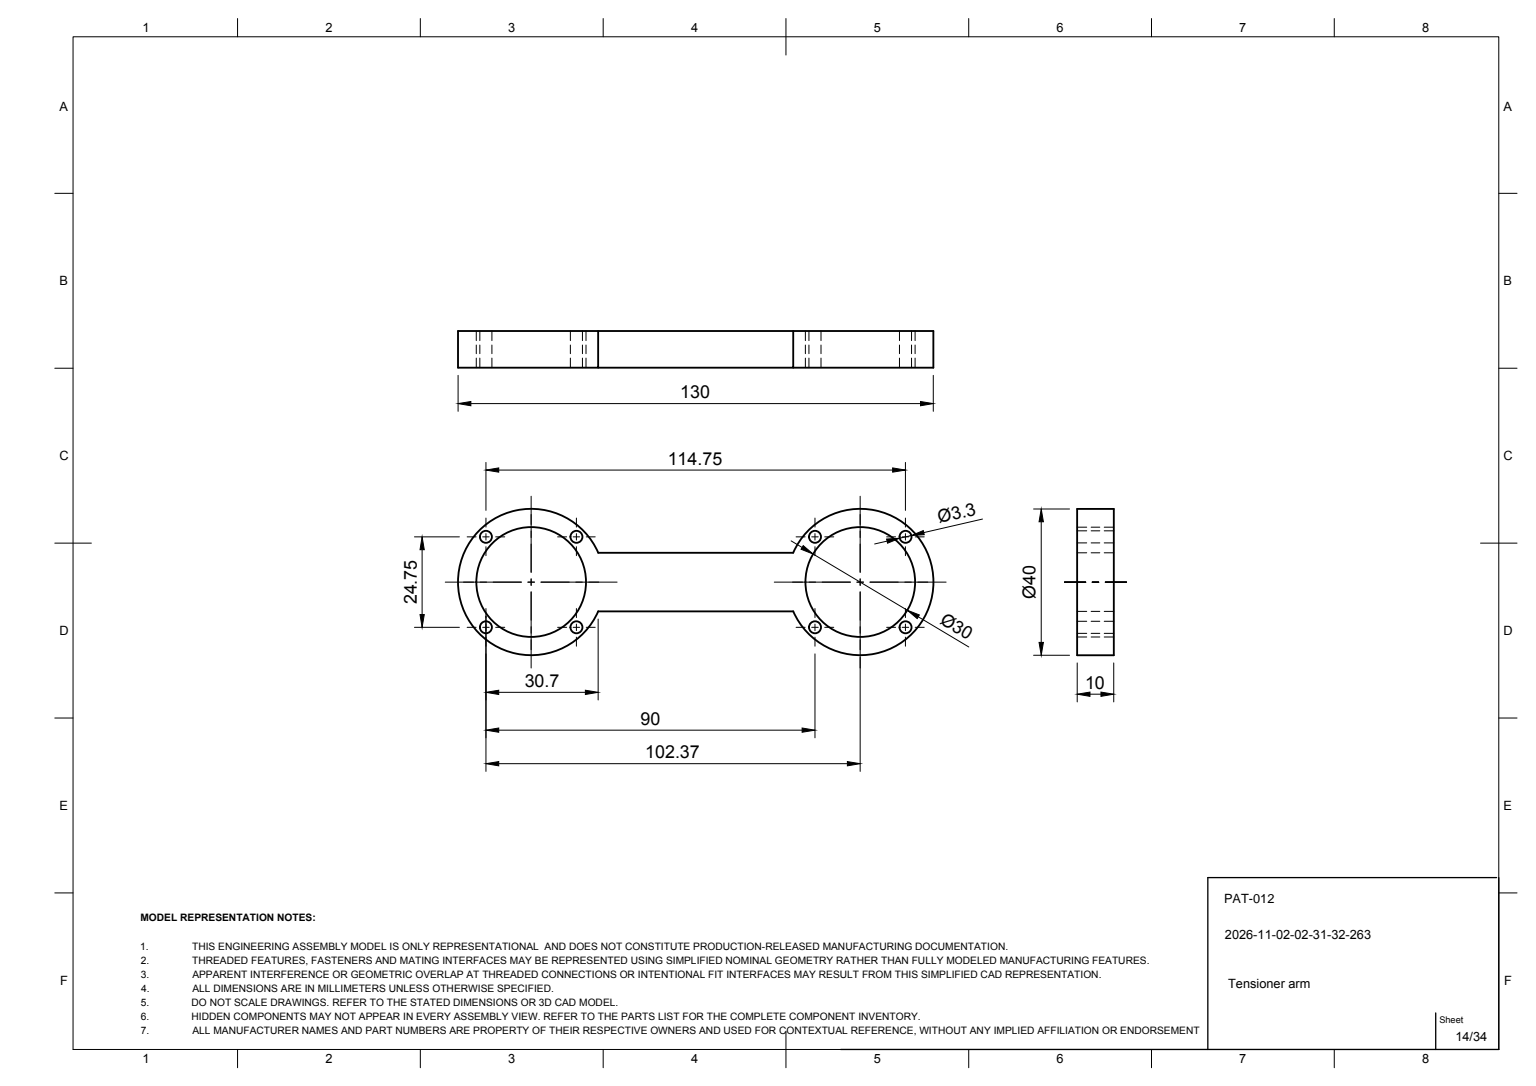
ISO-10303-21;
HEADER;
/* Generated by software containing ST-Developer
 * from STEP Tools, Inc. (www.steptools.com) 
 */

FILE_DESCRIPTION(
/* description */ ('Belt tensioner idler arm'),
/* implementation_level */ '2;1');

FILE_NAME(
/* name */ 'Tensioner arm.step',
/* time_stamp */ '2026-10-28T03:22:15-07:00',
/* author */ (''),
/* organization */ (''),
/* preprocessor_version */ 'ST-DEVELOPER v20.2',
/* originating_system */ 'Autodesk Translation Framework v15.17.0.0',
/* authorisation */ '');

FILE_SCHEMA (('AUTOMOTIVE_DESIGN { 1 0 10303 214 3 1 1 }'));
ENDSEC;

DATA;
#10=MECHANICAL_DESIGN_GEOMETRIC_PRESENTATION_REPRESENTATION('',(#459),#12779);
#391=SHAPE_REPRESENTATION_RELATIONSHIP('SRR','None',#12938,#425);
#425=ADVANCED_BREP_SHAPE_REPRESENTATION('',(#499),#12755);
#459=STYLED_ITEM('',(#13177),#499);
#499=MANIFOLD_SOLID_BREP('Body1',#6195);
#562=FACE_BOUND('',#1371,.T.);
#563=FACE_BOUND('',#1372,.T.);
#564=FACE_BOUND('',#1373,.T.);
#565=FACE_BOUND('',#1374,.T.);
#566=FACE_BOUND('',#1375,.T.);
#567=FACE_BOUND('',#1376,.T.);
#568=FACE_BOUND('',#1377,.T.);
#569=FACE_BOUND('',#1378,.T.);
#570=FACE_BOUND('',#1379,.T.);
#571=FACE_BOUND('',#1380,.T.);
#572=FACE_BOUND('',#1384,.T.);
#573=FACE_BOUND('',#1385,.T.);
#574=FACE_BOUND('',#1386,.T.);
#575=FACE_BOUND('',#1387,.T.);
#576=FACE_BOUND('',#1388,.T.);
#577=FACE_BOUND('',#1389,.T.);
#578=FACE_BOUND('',#1390,.T.);
#579=FACE_BOUND('',#1391,.T.);
#580=FACE_BOUND('',#1392,.T.);
#581=FACE_BOUND('',#1393,.T.);
#740=PLANE('',#6843);
#741=PLANE('',#6844);
#742=PLANE('',#6846);
#743=PLANE('',#6849);
#956=FACE_OUTER_BOUND('',#1358,.T.);
#957=FACE_OUTER_BOUND('',#1359,.T.);
#958=FACE_OUTER_BOUND('',#1360,.T.);
#959=FACE_OUTER_BOUND('',#1361,.T.);
#960=FACE_OUTER_BOUND('',#1362,.T.);
#961=FACE_OUTER_BOUND('',#1363,.T.);
#962=FACE_OUTER_BOUND('',#1364,.T.);
#963=FACE_OUTER_BOUND('',#1365,.T.);
#964=FACE_OUTER_BOUND('',#1366,.T.);
#965=FACE_OUTER_BOUND('',#1367,.T.);
#966=FACE_OUTER_BOUND('',#1368,.T.);
#967=FACE_OUTER_BOUND('',#1369,.T.);
#968=FACE_OUTER_BOUND('',#1370,.T.);
#969=FACE_OUTER_BOUND('',#1381,.T.);
#970=FACE_OUTER_BOUND('',#1382,.T.);
#971=FACE_OUTER_BOUND('',#1383,.T.);
#1358=EDGE_LOOP('',(#4554,#4555,#4556,#4557));
#1359=EDGE_LOOP('',(#4558,#4559,#4560,#4561));
#1360=EDGE_LOOP('',(#4562,#4563,#4564,#4565));
#1361=EDGE_LOOP('',(#4566,#4567,#4568,#4569));
#1362=EDGE_LOOP('',(#4570,#4571,#4572,#4573));
#1363=EDGE_LOOP('',(#4574,#4575,#4576,#4577));
#1364=EDGE_LOOP('',(#4578,#4579,#4580,#4581));
#1365=EDGE_LOOP('',(#4582,#4583,#4584,#4585));
#1366=EDGE_LOOP('',(#4586,#4587,#4588,#4589));
#1367=EDGE_LOOP('',(#4590,#4591,#4592,#4593));
#1368=EDGE_LOOP('',(#4594,#4595,#4596,#4597));
#1369=EDGE_LOOP('',(#4598,#4599,#4600,#4601));
#1370=EDGE_LOOP('',(#4602,#4603,#4604,#4605));
#1371=EDGE_LOOP('',(#4606));
#1372=EDGE_LOOP('',(#4607));
#1373=EDGE_LOOP('',(#4608));
#1374=EDGE_LOOP('',(#4609));
#1375=EDGE_LOOP('',(#4610));
#1376=EDGE_LOOP('',(#4611));
#1377=EDGE_LOOP('',(#4612));
#1378=EDGE_LOOP('',(#4613));
#1379=EDGE_LOOP('',(#4614));
#1380=EDGE_LOOP('',(#4615));
#1381=EDGE_LOOP('',(#4616,#4617,#4618,#4619));
#1382=EDGE_LOOP('',(#4620,#4621,#4622,#4623));
#1383=EDGE_LOOP('',(#4624,#4625,#4626,#4627));
#1384=EDGE_LOOP('',(#4628));
#1385=EDGE_LOOP('',(#4629));
#1386=EDGE_LOOP('',(#4630));
#1387=EDGE_LOOP('',(#4631));
#1388=EDGE_LOOP('',(#4632));
#1389=EDGE_LOOP('',(#4633));
#1390=EDGE_LOOP('',(#4634));
#1391=EDGE_LOOP('',(#4635));
#1392=EDGE_LOOP('',(#4636));
#1393=EDGE_LOOP('',(#4637));
#1843=LINE('',#10693,#2192);
#1844=LINE('',#10699,#2193);
#1845=LINE('',#10705,#2194);
#1846=LINE('',#10711,#2195);
#1847=LINE('',#10717,#2196);
#1848=LINE('',#10723,#2197);
#1849=LINE('',#10729,#2198);
#1850=LINE('',#10735,#2199);
#1851=LINE('',#10741,#2200);
#1852=LINE('',#10747,#2201);
#1853=LINE('',#10752,#2202);
#1854=LINE('',#10756,#2203);
#1855=LINE('',#10760,#2204);
#1856=LINE('',#10762,#2205);
#1857=LINE('',#10763,#2206);
#1858=LINE('',#10766,#2207);
#1859=LINE('',#10770,#2208);
#1860=LINE('',#10771,#2209);
#2192=VECTOR('',#7989,0.165);
#2193=VECTOR('',#7996,0.165);
#2194=VECTOR('',#8003,0.164999999999999);
#2195=VECTOR('',#8010,0.164999999999999);
#2196=VECTOR('',#8017,0.165);
#2197=VECTOR('',#8024,0.165);
#2198=VECTOR('',#8031,0.165);
#2199=VECTOR('',#8038,0.165);
#2200=VECTOR('',#8045,1.5);
#2201=VECTOR('',#8052,1.5);
#2202=VECTOR('',#8057,1.);
#2203=VECTOR('',#8060,1.);
#2204=VECTOR('',#8065,1.);
#2205=VECTOR('',#8066,1.);
#2206=VECTOR('',#8067,1.);
#2207=VECTOR('',#8070,1.);
#2208=VECTOR('',#8075,1.);
#2209=VECTOR('',#8076,1.);
#2478=CIRCLE('',#6811,0.165);
#2479=CIRCLE('',#6812,0.165);
#2480=CIRCLE('',#6814,0.165);
#2481=CIRCLE('',#6815,0.165);
#2482=CIRCLE('',#6817,0.164999999999999);
#2483=CIRCLE('',#6818,0.164999999999999);
#2484=CIRCLE('',#6820,0.164999999999999);
#2485=CIRCLE('',#6821,0.164999999999999);
#2486=CIRCLE('',#6823,0.165);
#2487=CIRCLE('',#6824,0.165);
#2488=CIRCLE('',#6826,0.165);
#2489=CIRCLE('',#6827,0.165);
#2490=CIRCLE('',#6829,0.165);
#2491=CIRCLE('',#6830,0.165);
#2492=CIRCLE('',#6832,0.165);
#2493=CIRCLE('',#6833,0.165);
#2494=CIRCLE('',#6835,1.5);
#2495=CIRCLE('',#6836,1.5);
#2496=CIRCLE('',#6838,1.5);
#2497=CIRCLE('',#6839,1.5);
#2498=CIRCLE('',#6841,2.);
#2499=CIRCLE('',#6842,2.);
#2500=CIRCLE('',#6845,2.);
#2501=CIRCLE('',#6848,2.);
#2919=VERTEX_POINT('',#10690);
#2920=VERTEX_POINT('',#10692);
#2921=VERTEX_POINT('',#10696);
#2922=VERTEX_POINT('',#10698);
#2923=VERTEX_POINT('',#10702);
#2924=VERTEX_POINT('',#10704);
#2925=VERTEX_POINT('',#10708);
#2926=VERTEX_POINT('',#10710);
#2927=VERTEX_POINT('',#10714);
#2928=VERTEX_POINT('',#10716);
#2929=VERTEX_POINT('',#10720);
#2930=VERTEX_POINT('',#10722);
#2931=VERTEX_POINT('',#10726);
#2932=VERTEX_POINT('',#10728);
#2933=VERTEX_POINT('',#10732);
#2934=VERTEX_POINT('',#10734);
#2935=VERTEX_POINT('',#10738);
#2936=VERTEX_POINT('',#10740);
#2937=VERTEX_POINT('',#10744);
#2938=VERTEX_POINT('',#10746);
#2939=VERTEX_POINT('',#10750);
#2940=VERTEX_POINT('',#10751);
#2941=VERTEX_POINT('',#10753);
#2942=VERTEX_POINT('',#10755);
#2943=VERTEX_POINT('',#10759);
#2944=VERTEX_POINT('',#10761);
#2945=VERTEX_POINT('',#10765);
#2946=VERTEX_POINT('',#10769);
#3532=EDGE_CURVE('',#2919,#2919,#2478,.T.);
#3533=EDGE_CURVE('',#2919,#2920,#1843,.T.);
#3534=EDGE_CURVE('',#2920,#2920,#2479,.T.);
#3535=EDGE_CURVE('',#2921,#2921,#2480,.T.);
#3536=EDGE_CURVE('',#2921,#2922,#1844,.T.);
#3537=EDGE_CURVE('',#2922,#2922,#2481,.T.);
#3538=EDGE_CURVE('',#2923,#2923,#2482,.T.);
#3539=EDGE_CURVE('',#2923,#2924,#1845,.T.);
#3540=EDGE_CURVE('',#2924,#2924,#2483,.T.);
#3541=EDGE_CURVE('',#2925,#2925,#2484,.T.);
#3542=EDGE_CURVE('',#2925,#2926,#1846,.T.);
#3543=EDGE_CURVE('',#2926,#2926,#2485,.T.);
#3544=EDGE_CURVE('',#2927,#2927,#2486,.T.);
#3545=EDGE_CURVE('',#2927,#2928,#1847,.T.);
#3546=EDGE_CURVE('',#2928,#2928,#2487,.T.);
#3547=EDGE_CURVE('',#2929,#2929,#2488,.T.);
#3548=EDGE_CURVE('',#2929,#2930,#1848,.T.);
#3549=EDGE_CURVE('',#2930,#2930,#2489,.T.);
#3550=EDGE_CURVE('',#2931,#2931,#2490,.T.);
#3551=EDGE_CURVE('',#2931,#2932,#1849,.T.);
#3552=EDGE_CURVE('',#2932,#2932,#2491,.T.);
#3553=EDGE_CURVE('',#2933,#2933,#2492,.T.);
#3554=EDGE_CURVE('',#2933,#2934,#1850,.T.);
#3555=EDGE_CURVE('',#2934,#2934,#2493,.T.);
#3556=EDGE_CURVE('',#2935,#2935,#2494,.T.);
#3557=EDGE_CURVE('',#2935,#2936,#1851,.T.);
#3558=EDGE_CURVE('',#2936,#2936,#2495,.T.);
#3559=EDGE_CURVE('',#2937,#2937,#2496,.T.);
#3560=EDGE_CURVE('',#2937,#2938,#1852,.T.);
#3561=EDGE_CURVE('',#2938,#2938,#2497,.T.);
#3562=EDGE_CURVE('',#2939,#2940,#1853,.T.);
#3563=EDGE_CURVE('',#2941,#2939,#2498,.T.);
#3564=EDGE_CURVE('',#2942,#2941,#1854,.T.);
#3565=EDGE_CURVE('',#2942,#2940,#2499,.T.);
#3566=EDGE_CURVE('',#2940,#2943,#1855,.T.);
#3567=EDGE_CURVE('',#2944,#2943,#1856,.T.);
#3568=EDGE_CURVE('',#2939,#2944,#1857,.T.);
#3569=EDGE_CURVE('',#2945,#2942,#1858,.T.);
#3570=EDGE_CURVE('',#2943,#2945,#2500,.T.);
#3571=EDGE_CURVE('',#2946,#2941,#1859,.T.);
#3572=EDGE_CURVE('',#2945,#2946,#1860,.T.);
#3573=EDGE_CURVE('',#2944,#2946,#2501,.T.);
#4554=ORIENTED_EDGE('',*,*,#3532,.F.);
#4555=ORIENTED_EDGE('',*,*,#3533,.T.);
#4556=ORIENTED_EDGE('',*,*,#3534,.F.);
#4557=ORIENTED_EDGE('',*,*,#3533,.F.);
#4558=ORIENTED_EDGE('',*,*,#3535,.F.);
#4559=ORIENTED_EDGE('',*,*,#3536,.T.);
#4560=ORIENTED_EDGE('',*,*,#3537,.F.);
#4561=ORIENTED_EDGE('',*,*,#3536,.F.);
#4562=ORIENTED_EDGE('',*,*,#3538,.F.);
#4563=ORIENTED_EDGE('',*,*,#3539,.T.);
#4564=ORIENTED_EDGE('',*,*,#3540,.F.);
#4565=ORIENTED_EDGE('',*,*,#3539,.F.);
#4566=ORIENTED_EDGE('',*,*,#3541,.F.);
#4567=ORIENTED_EDGE('',*,*,#3542,.T.);
#4568=ORIENTED_EDGE('',*,*,#3543,.F.);
#4569=ORIENTED_EDGE('',*,*,#3542,.F.);
#4570=ORIENTED_EDGE('',*,*,#3544,.F.);
#4571=ORIENTED_EDGE('',*,*,#3545,.T.);
#4572=ORIENTED_EDGE('',*,*,#3546,.F.);
#4573=ORIENTED_EDGE('',*,*,#3545,.F.);
#4574=ORIENTED_EDGE('',*,*,#3547,.F.);
#4575=ORIENTED_EDGE('',*,*,#3548,.T.);
#4576=ORIENTED_EDGE('',*,*,#3549,.F.);
#4577=ORIENTED_EDGE('',*,*,#3548,.F.);
#4578=ORIENTED_EDGE('',*,*,#3550,.F.);
#4579=ORIENTED_EDGE('',*,*,#3551,.T.);
#4580=ORIENTED_EDGE('',*,*,#3552,.F.);
#4581=ORIENTED_EDGE('',*,*,#3551,.F.);
#4582=ORIENTED_EDGE('',*,*,#3553,.F.);
#4583=ORIENTED_EDGE('',*,*,#3554,.T.);
#4584=ORIENTED_EDGE('',*,*,#3555,.F.);
#4585=ORIENTED_EDGE('',*,*,#3554,.F.);
#4586=ORIENTED_EDGE('',*,*,#3556,.F.);
#4587=ORIENTED_EDGE('',*,*,#3557,.T.);
#4588=ORIENTED_EDGE('',*,*,#3558,.F.);
#4589=ORIENTED_EDGE('',*,*,#3557,.F.);
#4590=ORIENTED_EDGE('',*,*,#3559,.F.);
#4591=ORIENTED_EDGE('',*,*,#3560,.T.);
#4592=ORIENTED_EDGE('',*,*,#3561,.F.);
#4593=ORIENTED_EDGE('',*,*,#3560,.F.);
#4594=ORIENTED_EDGE('',*,*,#3562,.F.);
#4595=ORIENTED_EDGE('',*,*,#3563,.F.);
#4596=ORIENTED_EDGE('',*,*,#3564,.F.);
#4597=ORIENTED_EDGE('',*,*,#3565,.T.);
#4598=ORIENTED_EDGE('',*,*,#3562,.T.);
#4599=ORIENTED_EDGE('',*,*,#3566,.T.);
#4600=ORIENTED_EDGE('',*,*,#3567,.F.);
#4601=ORIENTED_EDGE('',*,*,#3568,.F.);
#4602=ORIENTED_EDGE('',*,*,#3565,.F.);
#4603=ORIENTED_EDGE('',*,*,#3569,.F.);
#4604=ORIENTED_EDGE('',*,*,#3570,.F.);
#4605=ORIENTED_EDGE('',*,*,#3566,.F.);
#4606=ORIENTED_EDGE('',*,*,#3544,.T.);
#4607=ORIENTED_EDGE('',*,*,#3547,.T.);
#4608=ORIENTED_EDGE('',*,*,#3550,.T.);
#4609=ORIENTED_EDGE('',*,*,#3553,.T.);
#4610=ORIENTED_EDGE('',*,*,#3556,.T.);
#4611=ORIENTED_EDGE('',*,*,#3559,.T.);
#4612=ORIENTED_EDGE('',*,*,#3541,.T.);
#4613=ORIENTED_EDGE('',*,*,#3538,.T.);
#4614=ORIENTED_EDGE('',*,*,#3535,.T.);
#4615=ORIENTED_EDGE('',*,*,#3532,.T.);
#4616=ORIENTED_EDGE('',*,*,#3564,.T.);
#4617=ORIENTED_EDGE('',*,*,#3571,.F.);
#4618=ORIENTED_EDGE('',*,*,#3572,.F.);
#4619=ORIENTED_EDGE('',*,*,#3569,.T.);
#4620=ORIENTED_EDGE('',*,*,#3567,.T.);
#4621=ORIENTED_EDGE('',*,*,#3570,.T.);
#4622=ORIENTED_EDGE('',*,*,#3572,.T.);
#4623=ORIENTED_EDGE('',*,*,#3573,.F.);
#4624=ORIENTED_EDGE('',*,*,#3568,.T.);
#4625=ORIENTED_EDGE('',*,*,#3573,.T.);
#4626=ORIENTED_EDGE('',*,*,#3571,.T.);
#4627=ORIENTED_EDGE('',*,*,#3563,.T.);
#4628=ORIENTED_EDGE('',*,*,#3546,.T.);
#4629=ORIENTED_EDGE('',*,*,#3549,.T.);
#4630=ORIENTED_EDGE('',*,*,#3552,.T.);
#4631=ORIENTED_EDGE('',*,*,#3555,.T.);
#4632=ORIENTED_EDGE('',*,*,#3558,.T.);
#4633=ORIENTED_EDGE('',*,*,#3561,.T.);
#4634=ORIENTED_EDGE('',*,*,#3543,.T.);
#4635=ORIENTED_EDGE('',*,*,#3540,.T.);
#4636=ORIENTED_EDGE('',*,*,#3537,.T.);
#4637=ORIENTED_EDGE('',*,*,#3534,.T.);
#5692=CYLINDRICAL_SURFACE('',#6810,0.165);
#5693=CYLINDRICAL_SURFACE('',#6813,0.165);
#5694=CYLINDRICAL_SURFACE('',#6816,0.164999999999999);
#5695=CYLINDRICAL_SURFACE('',#6819,0.164999999999999);
#5696=CYLINDRICAL_SURFACE('',#6822,0.165);
#5697=CYLINDRICAL_SURFACE('',#6825,0.165);
#5698=CYLINDRICAL_SURFACE('',#6828,0.165);
#5699=CYLINDRICAL_SURFACE('',#6831,0.165);
#5700=CYLINDRICAL_SURFACE('',#6834,1.5);
#5701=CYLINDRICAL_SURFACE('',#6837,1.5);
#5702=CYLINDRICAL_SURFACE('',#6840,2.);
#5703=CYLINDRICAL_SURFACE('',#6847,2.);
#5933=ADVANCED_FACE('',(#956),#5692,.F.);
#5934=ADVANCED_FACE('',(#957),#5693,.F.);
#5935=ADVANCED_FACE('',(#958),#5694,.F.);
#5936=ADVANCED_FACE('',(#959),#5695,.F.);
#5937=ADVANCED_FACE('',(#960),#5696,.F.);
#5938=ADVANCED_FACE('',(#961),#5697,.F.);
#5939=ADVANCED_FACE('',(#962),#5698,.F.);
#5940=ADVANCED_FACE('',(#963),#5699,.F.);
#5941=ADVANCED_FACE('',(#964),#5700,.F.);
#5942=ADVANCED_FACE('',(#965),#5701,.F.);
#5943=ADVANCED_FACE('',(#966),#5702,.T.);
#5944=ADVANCED_FACE('',(#967),#740,.T.);
#5945=ADVANCED_FACE('',(#968,#562,#563,#564,#565,#566,#567,#568,#569,#570,
#571),#741,.F.);
#5946=ADVANCED_FACE('',(#969),#742,.T.);
#5947=ADVANCED_FACE('',(#970),#5703,.T.);
#5948=ADVANCED_FACE('',(#971,#572,#573,#574,#575,#576,#577,#578,#579,#580,
#581),#743,.T.);
#6195=CLOSED_SHELL('',(#5933,#5934,#5935,#5936,#5937,#5938,#5939,#5940,
#5941,#5942,#5943,#5944,#5945,#5946,#5947,#5948));
#6809=AXIS2_PLACEMENT_3D('',#10688,#7983,#7984);
#6810=AXIS2_PLACEMENT_3D('',#10689,#7985,#7986);
#6811=AXIS2_PLACEMENT_3D('',#10691,#7987,#7988);
#6812=AXIS2_PLACEMENT_3D('',#10694,#7990,#7991);
#6813=AXIS2_PLACEMENT_3D('',#10695,#7992,#7993);
#6814=AXIS2_PLACEMENT_3D('',#10697,#7994,#7995);
#6815=AXIS2_PLACEMENT_3D('',#10700,#7997,#7998);
#6816=AXIS2_PLACEMENT_3D('',#10701,#7999,#8000);
#6817=AXIS2_PLACEMENT_3D('',#10703,#8001,#8002);
#6818=AXIS2_PLACEMENT_3D('',#10706,#8004,#8005);
#6819=AXIS2_PLACEMENT_3D('',#10707,#8006,#8007);
#6820=AXIS2_PLACEMENT_3D('',#10709,#8008,#8009);
#6821=AXIS2_PLACEMENT_3D('',#10712,#8011,#8012);
#6822=AXIS2_PLACEMENT_3D('',#10713,#8013,#8014);
#6823=AXIS2_PLACEMENT_3D('',#10715,#8015,#8016);
#6824=AXIS2_PLACEMENT_3D('',#10718,#8018,#8019);
#6825=AXIS2_PLACEMENT_3D('',#10719,#8020,#8021);
#6826=AXIS2_PLACEMENT_3D('',#10721,#8022,#8023);
#6827=AXIS2_PLACEMENT_3D('',#10724,#8025,#8026);
#6828=AXIS2_PLACEMENT_3D('',#10725,#8027,#8028);
#6829=AXIS2_PLACEMENT_3D('',#10727,#8029,#8030);
#6830=AXIS2_PLACEMENT_3D('',#10730,#8032,#8033);
#6831=AXIS2_PLACEMENT_3D('',#10731,#8034,#8035);
#6832=AXIS2_PLACEMENT_3D('',#10733,#8036,#8037);
#6833=AXIS2_PLACEMENT_3D('',#10736,#8039,#8040);
#6834=AXIS2_PLACEMENT_3D('',#10737,#8041,#8042);
#6835=AXIS2_PLACEMENT_3D('',#10739,#8043,#8044);
#6836=AXIS2_PLACEMENT_3D('',#10742,#8046,#8047);
#6837=AXIS2_PLACEMENT_3D('',#10743,#8048,#8049);
#6838=AXIS2_PLACEMENT_3D('',#10745,#8050,#8051);
#6839=AXIS2_PLACEMENT_3D('',#10748,#8053,#8054);
#6840=AXIS2_PLACEMENT_3D('',#10749,#8055,#8056);
#6841=AXIS2_PLACEMENT_3D('',#10754,#8058,#8059);
#6842=AXIS2_PLACEMENT_3D('',#10757,#8061,#8062);
#6843=AXIS2_PLACEMENT_3D('',#10758,#8063,#8064);
#6844=AXIS2_PLACEMENT_3D('',#10764,#8068,#8069);
#6845=AXIS2_PLACEMENT_3D('',#10767,#8071,#8072);
#6846=AXIS2_PLACEMENT_3D('',#10768,#8073,#8074);
#6847=AXIS2_PLACEMENT_3D('',#10772,#8077,#8078);
#6848=AXIS2_PLACEMENT_3D('',#10773,#8079,#8080);
#6849=AXIS2_PLACEMENT_3D('',#10774,#8081,#8082);
#7983=DIRECTION('axis',(0.,0.,1.));
#7984=DIRECTION('refdir',(1.,0.,0.));
#7985=DIRECTION('center_axis',(0.,0.,1.));
#7986=DIRECTION('ref_axis',(1.,0.,0.));
#7987=DIRECTION('center_axis',(0.,0.,1.));
#7988=DIRECTION('ref_axis',(1.,0.,0.));
#7989=DIRECTION('',(0.,0.,1.));
#7990=DIRECTION('center_axis',(0.,0.,-1.));
#7991=DIRECTION('ref_axis',(1.,0.,0.));
#7992=DIRECTION('center_axis',(0.,0.,1.));
#7993=DIRECTION('ref_axis',(1.,0.,0.));
#7994=DIRECTION('center_axis',(0.,0.,1.));
#7995=DIRECTION('ref_axis',(1.,0.,0.));
#7996=DIRECTION('',(0.,0.,1.));
#7997=DIRECTION('center_axis',(0.,0.,-1.));
#7998=DIRECTION('ref_axis',(1.,0.,0.));
#7999=DIRECTION('center_axis',(0.,0.,1.));
#8000=DIRECTION('ref_axis',(1.,0.,0.));
#8001=DIRECTION('center_axis',(0.,0.,1.));
#8002=DIRECTION('ref_axis',(1.,0.,0.));
#8003=DIRECTION('',(0.,0.,1.));
#8004=DIRECTION('center_axis',(0.,0.,-1.));
#8005=DIRECTION('ref_axis',(1.,0.,0.));
#8006=DIRECTION('center_axis',(0.,0.,1.));
#8007=DIRECTION('ref_axis',(1.,0.,0.));
#8008=DIRECTION('center_axis',(0.,0.,1.));
#8009=DIRECTION('ref_axis',(1.,0.,0.));
#8010=DIRECTION('',(0.,0.,1.));
#8011=DIRECTION('center_axis',(0.,0.,-1.));
#8012=DIRECTION('ref_axis',(1.,0.,0.));
#8013=DIRECTION('center_axis',(0.,0.,1.));
#8014=DIRECTION('ref_axis',(1.,0.,0.));
#8015=DIRECTION('center_axis',(0.,0.,1.));
#8016=DIRECTION('ref_axis',(1.,0.,0.));
#8017=DIRECTION('',(0.,0.,1.));
#8018=DIRECTION('center_axis',(0.,0.,-1.));
#8019=DIRECTION('ref_axis',(1.,0.,0.));
#8020=DIRECTION('center_axis',(0.,0.,1.));
#8021=DIRECTION('ref_axis',(1.,0.,0.));
#8022=DIRECTION('center_axis',(0.,0.,1.));
#8023=DIRECTION('ref_axis',(1.,0.,0.));
#8024=DIRECTION('',(0.,0.,1.));
#8025=DIRECTION('center_axis',(0.,0.,-1.));
#8026=DIRECTION('ref_axis',(1.,0.,0.));
#8027=DIRECTION('center_axis',(0.,0.,1.));
#8028=DIRECTION('ref_axis',(1.,0.,0.));
#8029=DIRECTION('center_axis',(0.,0.,1.));
#8030=DIRECTION('ref_axis',(1.,0.,0.));
#8031=DIRECTION('',(0.,0.,1.));
#8032=DIRECTION('center_axis',(0.,0.,-1.));
#8033=DIRECTION('ref_axis',(1.,0.,0.));
#8034=DIRECTION('center_axis',(0.,0.,1.));
#8035=DIRECTION('ref_axis',(1.,0.,0.));
#8036=DIRECTION('center_axis',(0.,0.,1.));
#8037=DIRECTION('ref_axis',(1.,0.,0.));
#8038=DIRECTION('',(0.,0.,1.));
#8039=DIRECTION('center_axis',(0.,0.,-1.));
#8040=DIRECTION('ref_axis',(1.,0.,0.));
#8041=DIRECTION('center_axis',(0.,0.,1.));
#8042=DIRECTION('ref_axis',(1.,0.,0.));
#8043=DIRECTION('center_axis',(0.,0.,1.));
#8044=DIRECTION('ref_axis',(1.,0.,0.));
#8045=DIRECTION('',(0.,0.,1.));
#8046=DIRECTION('center_axis',(0.,0.,-1.));
#8047=DIRECTION('ref_axis',(1.,0.,0.));
#8048=DIRECTION('center_axis',(0.,0.,1.));
#8049=DIRECTION('ref_axis',(1.,0.,0.));
#8050=DIRECTION('center_axis',(0.,0.,1.));
#8051=DIRECTION('ref_axis',(1.,0.,0.));
#8052=DIRECTION('',(0.,0.,1.));
#8053=DIRECTION('center_axis',(0.,0.,-1.));
#8054=DIRECTION('ref_axis',(1.,0.,0.));
#8055=DIRECTION('center_axis',(0.,0.,1.));
#8056=DIRECTION('ref_axis',(1.,0.,0.));
#8057=DIRECTION('',(0.,0.,-1.));
#8058=DIRECTION('center_axis',(0.,0.,1.));
#8059=DIRECTION('ref_axis',(1.,0.,0.));
#8060=DIRECTION('',(0.,0.,1.));
#8061=DIRECTION('center_axis',(0.,0.,1.));
#8062=DIRECTION('ref_axis',(1.,0.,0.));
#8063=DIRECTION('center_axis',(0.,1.,0.));
#8064=DIRECTION('ref_axis',(-1.,0.,0.));
#8065=DIRECTION('',(-1.,0.,0.));
#8066=DIRECTION('',(0.,0.,-1.));
#8067=DIRECTION('',(-1.,0.,0.));
#8068=DIRECTION('center_axis',(0.,0.,1.));
#8069=DIRECTION('ref_axis',(1.,0.,0.));
#8070=DIRECTION('',(1.,0.,0.));
#8071=DIRECTION('center_axis',(0.,0.,1.));
#8072=DIRECTION('ref_axis',(1.,0.,0.));
#8073=DIRECTION('center_axis',(0.,-1.,0.));
#8074=DIRECTION('ref_axis',(1.,0.,0.));
#8075=DIRECTION('',(1.,0.,0.));
#8076=DIRECTION('',(0.,0.,1.));
#8077=DIRECTION('center_axis',(0.,0.,1.));
#8078=DIRECTION('ref_axis',(-1.,1.22464679914735E-16,0.));
#8079=DIRECTION('center_axis',(0.,0.,1.));
#8080=DIRECTION('ref_axis',(1.,0.,0.));
#8081=DIRECTION('center_axis',(0.,0.,1.));
#8082=DIRECTION('ref_axis',(1.,0.,0.));
#10688=CARTESIAN_POINT('',(0.,0.,0.));
#10689=CARTESIAN_POINT('Origin',(7.76256313292354,-1.23743686707646,4.9));
#10690=CARTESIAN_POINT('',(7.59756313292354,-1.23743686707646,5.));
#10691=CARTESIAN_POINT('Origin',(7.76256313292354,-1.23743686707646,5.));
#10692=CARTESIAN_POINT('',(7.59756313292354,-1.23743686707646,6.));
#10693=CARTESIAN_POINT('',(7.59756313292354,-1.23743686707646,4.9));
#10694=CARTESIAN_POINT('Origin',(7.76256313292354,-1.23743686707646,6.));
#10695=CARTESIAN_POINT('Origin',(7.76256313292354,1.23743686707646,4.9));
#10696=CARTESIAN_POINT('',(7.59756313292354,1.23743686707646,5.));
#10697=CARTESIAN_POINT('Origin',(7.76256313292354,1.23743686707646,5.));
#10698=CARTESIAN_POINT('',(7.59756313292354,1.23743686707646,6.));
#10699=CARTESIAN_POINT('',(7.59756313292354,1.23743686707646,4.9));
#10700=CARTESIAN_POINT('Origin',(7.76256313292354,1.23743686707646,6.));
#10701=CARTESIAN_POINT('Origin',(10.2374368670765,1.23743686707646,4.9));
#10702=CARTESIAN_POINT('',(10.0724368670765,1.23743686707646,5.));
#10703=CARTESIAN_POINT('Origin',(10.2374368670765,1.23743686707646,5.));
#10704=CARTESIAN_POINT('',(10.0724368670765,1.23743686707646,6.));
#10705=CARTESIAN_POINT('',(10.0724368670765,1.23743686707646,4.9));
#10706=CARTESIAN_POINT('Origin',(10.2374368670765,1.23743686707646,6.));
#10707=CARTESIAN_POINT('Origin',(10.2374368670765,-1.23743686707646,4.9));
#10708=CARTESIAN_POINT('',(10.0724368670765,-1.23743686707646,5.));
#10709=CARTESIAN_POINT('Origin',(10.2374368670765,-1.23743686707646,5.));
#10710=CARTESIAN_POINT('',(10.0724368670765,-1.23743686707646,6.));
#10711=CARTESIAN_POINT('',(10.0724368670765,-1.23743686707646,4.9));
#10712=CARTESIAN_POINT('Origin',(10.2374368670765,-1.23743686707646,6.));
#10713=CARTESIAN_POINT('Origin',(-1.23743686707646,-1.23743686707646,4.9));
#10714=CARTESIAN_POINT('',(-1.40243686707646,-1.23743686707646,5.));
#10715=CARTESIAN_POINT('Origin',(-1.23743686707646,-1.23743686707646,5.));
#10716=CARTESIAN_POINT('',(-1.40243686707646,-1.23743686707646,6.));
#10717=CARTESIAN_POINT('',(-1.40243686707646,-1.23743686707646,4.9));
#10718=CARTESIAN_POINT('Origin',(-1.23743686707646,-1.23743686707646,6.));
#10719=CARTESIAN_POINT('Origin',(-1.23743686707646,1.23743686707646,4.9));
#10720=CARTESIAN_POINT('',(-1.40243686707646,1.23743686707646,5.));
#10721=CARTESIAN_POINT('Origin',(-1.23743686707646,1.23743686707646,5.));
#10722=CARTESIAN_POINT('',(-1.40243686707646,1.23743686707646,6.));
#10723=CARTESIAN_POINT('',(-1.40243686707646,1.23743686707646,4.9));
#10724=CARTESIAN_POINT('Origin',(-1.23743686707646,1.23743686707646,6.));
#10725=CARTESIAN_POINT('Origin',(1.23743686707646,1.23743686707646,4.9));
#10726=CARTESIAN_POINT('',(1.07243686707646,1.23743686707646,5.));
#10727=CARTESIAN_POINT('Origin',(1.23743686707646,1.23743686707646,5.));
#10728=CARTESIAN_POINT('',(1.07243686707646,1.23743686707646,6.));
#10729=CARTESIAN_POINT('',(1.07243686707646,1.23743686707646,4.9));
#10730=CARTESIAN_POINT('Origin',(1.23743686707646,1.23743686707646,6.));
#10731=CARTESIAN_POINT('Origin',(1.23743686707646,-1.23743686707646,4.9));
#10732=CARTESIAN_POINT('',(1.07243686707646,-1.23743686707646,5.));
#10733=CARTESIAN_POINT('Origin',(1.23743686707646,-1.23743686707646,5.));
#10734=CARTESIAN_POINT('',(1.07243686707646,-1.23743686707646,6.));
#10735=CARTESIAN_POINT('',(1.07243686707646,-1.23743686707646,4.9));
#10736=CARTESIAN_POINT('Origin',(1.23743686707646,-1.23743686707646,6.));
#10737=CARTESIAN_POINT('Origin',(0.,0.,4.9));
#10738=CARTESIAN_POINT('',(-1.5,-1.83697019872103E-16,5.));
#10739=CARTESIAN_POINT('Origin',(0.,0.,5.));
#10740=CARTESIAN_POINT('',(-1.5,1.83697019872103E-16,6.));
#10741=CARTESIAN_POINT('',(-1.5,-1.83697019872103E-16,4.9));
#10742=CARTESIAN_POINT('Origin',(0.,0.,6.));
#10743=CARTESIAN_POINT('Origin',(9.,0.,4.9));
#10744=CARTESIAN_POINT('',(7.5,-1.83697019872103E-16,5.));
#10745=CARTESIAN_POINT('Origin',(9.,0.,5.));
#10746=CARTESIAN_POINT('',(7.5,1.83697019872103E-16,6.));
#10747=CARTESIAN_POINT('',(7.5,-1.83697019872103E-16,4.9));
#10748=CARTESIAN_POINT('Origin',(9.,0.,6.));
#10749=CARTESIAN_POINT('Origin',(9.,0.,5.));
#10750=CARTESIAN_POINT('',(7.16696972201766,0.8,6.));
#10751=CARTESIAN_POINT('',(7.16696972201766,0.8,5.));
#10752=CARTESIAN_POINT('',(7.16696972201766,0.8,5.));
#10753=CARTESIAN_POINT('',(7.16696972201766,-0.8,6.));
#10754=CARTESIAN_POINT('Origin',(9.,0.,6.));
#10755=CARTESIAN_POINT('',(7.16696972201766,-0.8,5.));
#10756=CARTESIAN_POINT('',(7.16696972201766,-0.8,5.));
#10757=CARTESIAN_POINT('Origin',(9.,0.,5.));
#10758=CARTESIAN_POINT('Origin',(9.,0.8,5.));
#10759=CARTESIAN_POINT('',(1.83303027798234,0.8,5.));
#10760=CARTESIAN_POINT('',(9.,0.8,5.));
#10761=CARTESIAN_POINT('',(1.83303027798234,0.8,6.));
#10762=CARTESIAN_POINT('',(1.83303027798234,0.8,5.));
#10763=CARTESIAN_POINT('',(9.,0.8,6.));
#10764=CARTESIAN_POINT('Origin',(0.,0.,5.));
#10765=CARTESIAN_POINT('',(1.83303027798234,-0.8,5.));
#10766=CARTESIAN_POINT('',(0.,-0.8,5.));
#10767=CARTESIAN_POINT('Origin',(0.,0.,5.));
#10768=CARTESIAN_POINT('Origin',(0.,-0.8,5.));
#10769=CARTESIAN_POINT('',(1.83303027798234,-0.8,6.));
#10770=CARTESIAN_POINT('',(0.,-0.8,6.));
#10771=CARTESIAN_POINT('',(1.83303027798234,-0.8,5.));
#10772=CARTESIAN_POINT('Origin',(0.,0.,5.));
#10773=CARTESIAN_POINT('Origin',(0.,0.,6.));
#10774=CARTESIAN_POINT('Origin',(0.,0.,6.));
#12715=UNCERTAINTY_MEASURE_WITH_UNIT(LENGTH_MEASURE(0.001),#12780,
'DISTANCE_ACCURACY_VALUE',
'Maximum model space distance between geometric entities at asserted c
onnectivities');
#12739=UNCERTAINTY_MEASURE_WITH_UNIT(LENGTH_MEASURE(0.001),#12780,
'DISTANCE_ACCURACY_VALUE',
'Maximum model space distance between geometric entities at asserted c
onnectivities');
#12755=(
GEOMETRIC_REPRESENTATION_CONTEXT(3)
GLOBAL_UNCERTAINTY_ASSIGNED_CONTEXT((#12715))
GLOBAL_UNIT_ASSIGNED_CONTEXT((#12780,#12782,#12783))
REPRESENTATION_CONTEXT('','3D')
);
#12779=(
GEOMETRIC_REPRESENTATION_CONTEXT(3)
GLOBAL_UNCERTAINTY_ASSIGNED_CONTEXT((#12739))
GLOBAL_UNIT_ASSIGNED_CONTEXT((#12780,#12782,#12783))
REPRESENTATION_CONTEXT('','3D')
);
#12780=(
LENGTH_UNIT()
NAMED_UNIT(*)
SI_UNIT(.CENTI.,.METRE.)
);
#12782=(
NAMED_UNIT(*)
PLANE_ANGLE_UNIT()
SI_UNIT($,.RADIAN.)
);
#12783=(
NAMED_UNIT(*)
SI_UNIT($,.STERADIAN.)
SOLID_ANGLE_UNIT()
);
#12799=SHAPE_DEFINITION_REPRESENTATION(#12838,#12938);
#12838=PRODUCT_DEFINITION_SHAPE('',$,#12978);
#12938=SHAPE_REPRESENTATION('',(#6809),#12755);
#12962=PRODUCT_DEFINITION_CONTEXT('part definition',#13081,'design');
#12978=PRODUCT_DEFINITION('Tensioner arm','Tensioner arm',#13017,#12962);
#13017=PRODUCT_DEFINITION_FORMATION('',$,#13098);
#13081=APPLICATION_CONTEXT(
'Core Data for Automotive Mechanical Design Process');
#13082=PRODUCT_CONTEXT('part definition',#13081,'mechanical');
#13098=PRODUCT('Tensioner arm','Tensioner arm','Tensioner arm',(#13082));
#13171=COLOUR_RGB('Sky Blue',0.24,0.69,0.87);
#13172=FILL_AREA_STYLE_COLOUR('',#13171);
#13173=FILL_AREA_STYLE('',(#13172));
#13174=SURFACE_STYLE_FILL_AREA(#13173);
#13175=SURFACE_SIDE_STYLE('',(#13174));
#13176=SURFACE_STYLE_USAGE(.BOTH.,#13175);
#13177=PRESENTATION_STYLE_ASSIGNMENT((#13176));
ENDSEC;
END-ISO-10303-21;
